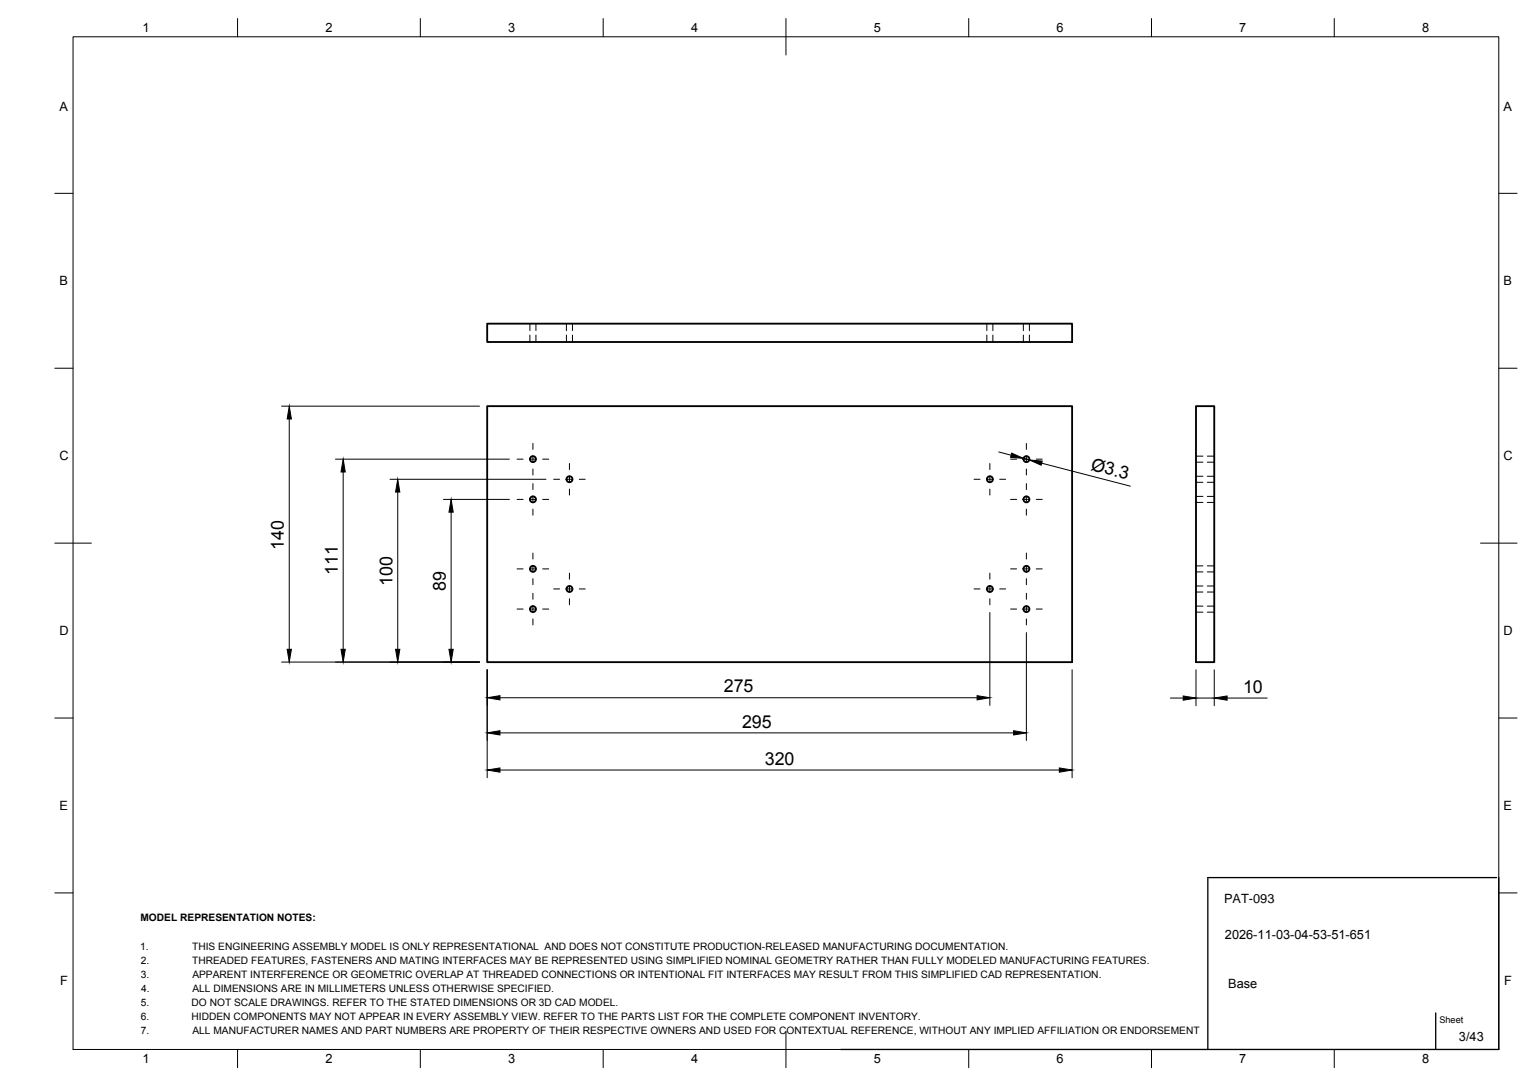
ISO-10303-21;
HEADER;
/* Generated by software containing ST-Developer
 * from STEP Tools, Inc. (www.steptools.com) 
 */

FILE_DESCRIPTION(
/* description */ ('Self-centering screw clamp'),
/* implementation_level */ '2;1');

FILE_NAME(
/* name */ 'Base.step',
/* time_stamp */ '2026-10-28T03:25:31-07:00',
/* author */ (''),
/* organization */ (''),
/* preprocessor_version */ 'ST-DEVELOPER v20.2',
/* originating_system */ 'Autodesk Translation Framework v15.17.0.0',
/* authorisation */ '');

FILE_SCHEMA (('AUTOMOTIVE_DESIGN { 1 0 10303 214 3 1 1 }'));
ENDSEC;

DATA;
#10=MECHANICAL_DESIGN_GEOMETRIC_PRESENTATION_REPRESENTATION('',(#624),#16799);
#542=SHAPE_REPRESENTATION_RELATIONSHIP('SRR','None',#17015,#583);
#583=ADVANCED_BREP_SHAPE_REPRESENTATION('',(#672),#16753);
#624=STYLED_ITEM('',(#17305),#672);
#672=MANIFOLD_SOLID_BREP('Body1',#9075);
#718=FACE_BOUND('',#1794,.T.);
#719=FACE_BOUND('',#1795,.T.);
#720=FACE_BOUND('',#1796,.T.);
#721=FACE_BOUND('',#1797,.T.);
#722=FACE_BOUND('',#1798,.T.);
#723=FACE_BOUND('',#1799,.T.);
#724=FACE_BOUND('',#1800,.T.);
#725=FACE_BOUND('',#1801,.T.);
#726=FACE_BOUND('',#1802,.T.);
#727=FACE_BOUND('',#1803,.T.);
#728=FACE_BOUND('',#1804,.T.);
#729=FACE_BOUND('',#1805,.T.);
#730=FACE_BOUND('',#1807,.T.);
#731=FACE_BOUND('',#1808,.T.);
#732=FACE_BOUND('',#1809,.T.);
#733=FACE_BOUND('',#1810,.T.);
#734=FACE_BOUND('',#1811,.T.);
#735=FACE_BOUND('',#1812,.T.);
#736=FACE_BOUND('',#1813,.T.);
#737=FACE_BOUND('',#1814,.T.);
#738=FACE_BOUND('',#1815,.T.);
#739=FACE_BOUND('',#1816,.T.);
#740=FACE_BOUND('',#1817,.T.);
#741=FACE_BOUND('',#1818,.T.);
#1014=PLANE('',#9616);
#1015=PLANE('',#9617);
#1016=PLANE('',#9618);
#1017=PLANE('',#9619);
#1018=PLANE('',#9620);
#1019=PLANE('',#9621);
#1273=FACE_OUTER_BOUND('',#1777,.T.);
#1274=FACE_OUTER_BOUND('',#1778,.T.);
#1275=FACE_OUTER_BOUND('',#1779,.T.);
#1276=FACE_OUTER_BOUND('',#1780,.T.);
#1277=FACE_OUTER_BOUND('',#1781,.T.);
#1278=FACE_OUTER_BOUND('',#1782,.T.);
#1279=FACE_OUTER_BOUND('',#1783,.T.);
#1280=FACE_OUTER_BOUND('',#1784,.T.);
#1281=FACE_OUTER_BOUND('',#1785,.T.);
#1282=FACE_OUTER_BOUND('',#1786,.T.);
#1283=FACE_OUTER_BOUND('',#1787,.T.);
#1284=FACE_OUTER_BOUND('',#1788,.T.);
#1285=FACE_OUTER_BOUND('',#1789,.T.);
#1286=FACE_OUTER_BOUND('',#1790,.T.);
#1287=FACE_OUTER_BOUND('',#1791,.T.);
#1288=FACE_OUTER_BOUND('',#1792,.T.);
#1289=FACE_OUTER_BOUND('',#1793,.T.);
#1290=FACE_OUTER_BOUND('',#1806,.T.);
#1777=EDGE_LOOP('',(#6103,#6104,#6105,#6106));
#1778=EDGE_LOOP('',(#6107,#6108,#6109,#6110));
#1779=EDGE_LOOP('',(#6111,#6112,#6113,#6114));
#1780=EDGE_LOOP('',(#6115,#6116,#6117,#6118));
#1781=EDGE_LOOP('',(#6119,#6120,#6121,#6122));
#1782=EDGE_LOOP('',(#6123,#6124,#6125,#6126));
#1783=EDGE_LOOP('',(#6127,#6128,#6129,#6130));
#1784=EDGE_LOOP('',(#6131,#6132,#6133,#6134));
#1785=EDGE_LOOP('',(#6135,#6136,#6137,#6138));
#1786=EDGE_LOOP('',(#6139,#6140,#6141,#6142));
#1787=EDGE_LOOP('',(#6143,#6144,#6145,#6146));
#1788=EDGE_LOOP('',(#6147,#6148,#6149,#6150));
#1789=EDGE_LOOP('',(#6151,#6152,#6153,#6154));
#1790=EDGE_LOOP('',(#6155,#6156,#6157,#6158));
#1791=EDGE_LOOP('',(#6159,#6160,#6161,#6162));
#1792=EDGE_LOOP('',(#6163,#6164,#6165,#6166));
#1793=EDGE_LOOP('',(#6167,#6168,#6169,#6170));
#1794=EDGE_LOOP('',(#6171));
#1795=EDGE_LOOP('',(#6172));
#1796=EDGE_LOOP('',(#6173));
#1797=EDGE_LOOP('',(#6174));
#1798=EDGE_LOOP('',(#6175));
#1799=EDGE_LOOP('',(#6176));
#1800=EDGE_LOOP('',(#6177));
#1801=EDGE_LOOP('',(#6178));
#1802=EDGE_LOOP('',(#6179));
#1803=EDGE_LOOP('',(#6180));
#1804=EDGE_LOOP('',(#6181));
#1805=EDGE_LOOP('',(#6182));
#1806=EDGE_LOOP('',(#6183,#6184,#6185,#6186));
#1807=EDGE_LOOP('',(#6187));
#1808=EDGE_LOOP('',(#6188));
#1809=EDGE_LOOP('',(#6189));
#1810=EDGE_LOOP('',(#6190));
#1811=EDGE_LOOP('',(#6191));
#1812=EDGE_LOOP('',(#6192));
#1813=EDGE_LOOP('',(#6193));
#1814=EDGE_LOOP('',(#6194));
#1815=EDGE_LOOP('',(#6195));
#1816=EDGE_LOOP('',(#6196));
#1817=EDGE_LOOP('',(#6197));
#1818=EDGE_LOOP('',(#6198));
#2577=LINE('',#13682,#3150);
#2578=LINE('',#13688,#3151);
#2579=LINE('',#13694,#3152);
#2580=LINE('',#13700,#3153);
#2581=LINE('',#13706,#3154);
#2582=LINE('',#13712,#3155);
#2583=LINE('',#13718,#3156);
#2584=LINE('',#13724,#3157);
#2585=LINE('',#13730,#3158);
#2586=LINE('',#13736,#3159);
#2587=LINE('',#13742,#3160);
#2588=LINE('',#13748,#3161);
#2589=LINE('',#13753,#3162);
#2590=LINE('',#13755,#3163);
#2591=LINE('',#13757,#3164);
#2592=LINE('',#13758,#3165);
#2593=LINE('',#13761,#3166);
#2594=LINE('',#13763,#3167);
#2595=LINE('',#13764,#3168);
#2596=LINE('',#13767,#3169);
#2597=LINE('',#13769,#3170);
#2598=LINE('',#13770,#3171);
#2599=LINE('',#13772,#3172);
#2600=LINE('',#13773,#3173);
#3150=VECTOR('',#10762,0.164999999999999);
#3151=VECTOR('',#10769,0.164999999999999);
#3152=VECTOR('',#10776,0.164999999999999);
#3153=VECTOR('',#10783,0.164999999999999);
#3154=VECTOR('',#10790,0.164999999999999);
#3155=VECTOR('',#10797,0.164999999999999);
#3156=VECTOR('',#10804,0.164999999999999);
#3157=VECTOR('',#10811,0.164999999999999);
#3158=VECTOR('',#10818,0.164999999999999);
#3159=VECTOR('',#10825,0.164999999999999);
#3160=VECTOR('',#10832,0.164999999999999);
#3161=VECTOR('',#10839,0.164999999999999);
#3162=VECTOR('',#10844,1.);
#3163=VECTOR('',#10845,1.);
#3164=VECTOR('',#10846,1.);
#3165=VECTOR('',#10847,1.);
#3166=VECTOR('',#10850,1.);
#3167=VECTOR('',#10851,1.);
#3168=VECTOR('',#10852,1.);
#3169=VECTOR('',#10855,1.);
#3170=VECTOR('',#10856,1.);
#3171=VECTOR('',#10857,1.);
#3172=VECTOR('',#10860,1.);
#3173=VECTOR('',#10861,1.);
#3723=CIRCLE('',#9581,0.164999999999999);
#3724=CIRCLE('',#9582,0.164999999999999);
#3725=CIRCLE('',#9584,0.164999999999999);
#3726=CIRCLE('',#9585,0.164999999999999);
#3727=CIRCLE('',#9587,0.164999999999999);
#3728=CIRCLE('',#9588,0.164999999999999);
#3729=CIRCLE('',#9590,0.164999999999999);
#3730=CIRCLE('',#9591,0.164999999999999);
#3731=CIRCLE('',#9593,0.164999999999999);
#3732=CIRCLE('',#9594,0.164999999999999);
#3733=CIRCLE('',#9596,0.164999999999999);
#3734=CIRCLE('',#9597,0.164999999999999);
#3735=CIRCLE('',#9599,0.164999999999999);
#3736=CIRCLE('',#9600,0.164999999999999);
#3737=CIRCLE('',#9602,0.164999999999999);
#3738=CIRCLE('',#9603,0.164999999999999);
#3739=CIRCLE('',#9605,0.164999999999999);
#3740=CIRCLE('',#9606,0.164999999999999);
#3741=CIRCLE('',#9608,0.164999999999999);
#3742=CIRCLE('',#9609,0.164999999999999);
#3743=CIRCLE('',#9611,0.164999999999999);
#3744=CIRCLE('',#9612,0.164999999999999);
#3745=CIRCLE('',#9614,0.164999999999999);
#3746=CIRCLE('',#9615,0.164999999999999);
#4233=VERTEX_POINT('',#13679);
#4234=VERTEX_POINT('',#13681);
#4235=VERTEX_POINT('',#13685);
#4236=VERTEX_POINT('',#13687);
#4237=VERTEX_POINT('',#13691);
#4238=VERTEX_POINT('',#13693);
#4239=VERTEX_POINT('',#13697);
#4240=VERTEX_POINT('',#13699);
#4241=VERTEX_POINT('',#13703);
#4242=VERTEX_POINT('',#13705);
#4243=VERTEX_POINT('',#13709);
#4244=VERTEX_POINT('',#13711);
#4245=VERTEX_POINT('',#13715);
#4246=VERTEX_POINT('',#13717);
#4247=VERTEX_POINT('',#13721);
#4248=VERTEX_POINT('',#13723);
#4249=VERTEX_POINT('',#13727);
#4250=VERTEX_POINT('',#13729);
#4251=VERTEX_POINT('',#13733);
#4252=VERTEX_POINT('',#13735);
#4253=VERTEX_POINT('',#13739);
#4254=VERTEX_POINT('',#13741);
#4255=VERTEX_POINT('',#13745);
#4256=VERTEX_POINT('',#13747);
#4257=VERTEX_POINT('',#13751);
#4258=VERTEX_POINT('',#13752);
#4259=VERTEX_POINT('',#13754);
#4260=VERTEX_POINT('',#13756);
#4261=VERTEX_POINT('',#13760);
#4262=VERTEX_POINT('',#13762);
#4263=VERTEX_POINT('',#13766);
#4264=VERTEX_POINT('',#13768);
#4976=EDGE_CURVE('',#4233,#4233,#3723,.T.);
#4977=EDGE_CURVE('',#4233,#4234,#2577,.T.);
#4978=EDGE_CURVE('',#4234,#4234,#3724,.T.);
#4979=EDGE_CURVE('',#4235,#4235,#3725,.T.);
#4980=EDGE_CURVE('',#4235,#4236,#2578,.T.);
#4981=EDGE_CURVE('',#4236,#4236,#3726,.T.);
#4982=EDGE_CURVE('',#4237,#4237,#3727,.T.);
#4983=EDGE_CURVE('',#4237,#4238,#2579,.T.);
#4984=EDGE_CURVE('',#4238,#4238,#3728,.T.);
#4985=EDGE_CURVE('',#4239,#4239,#3729,.T.);
#4986=EDGE_CURVE('',#4239,#4240,#2580,.T.);
#4987=EDGE_CURVE('',#4240,#4240,#3730,.T.);
#4988=EDGE_CURVE('',#4241,#4241,#3731,.T.);
#4989=EDGE_CURVE('',#4241,#4242,#2581,.T.);
#4990=EDGE_CURVE('',#4242,#4242,#3732,.T.);
#4991=EDGE_CURVE('',#4243,#4243,#3733,.T.);
#4992=EDGE_CURVE('',#4243,#4244,#2582,.T.);
#4993=EDGE_CURVE('',#4244,#4244,#3734,.T.);
#4994=EDGE_CURVE('',#4245,#4245,#3735,.T.);
#4995=EDGE_CURVE('',#4245,#4246,#2583,.T.);
#4996=EDGE_CURVE('',#4246,#4246,#3736,.T.);
#4997=EDGE_CURVE('',#4247,#4247,#3737,.T.);
#4998=EDGE_CURVE('',#4247,#4248,#2584,.T.);
#4999=EDGE_CURVE('',#4248,#4248,#3738,.T.);
#5000=EDGE_CURVE('',#4249,#4249,#3739,.T.);
#5001=EDGE_CURVE('',#4249,#4250,#2585,.T.);
#5002=EDGE_CURVE('',#4250,#4250,#3740,.T.);
#5003=EDGE_CURVE('',#4251,#4251,#3741,.T.);
#5004=EDGE_CURVE('',#4251,#4252,#2586,.T.);
#5005=EDGE_CURVE('',#4252,#4252,#3742,.T.);
#5006=EDGE_CURVE('',#4253,#4253,#3743,.T.);
#5007=EDGE_CURVE('',#4253,#4254,#2587,.T.);
#5008=EDGE_CURVE('',#4254,#4254,#3744,.T.);
#5009=EDGE_CURVE('',#4255,#4255,#3745,.T.);
#5010=EDGE_CURVE('',#4255,#4256,#2588,.T.);
#5011=EDGE_CURVE('',#4256,#4256,#3746,.T.);
#5012=EDGE_CURVE('',#4257,#4258,#2589,.T.);
#5013=EDGE_CURVE('',#4258,#4259,#2590,.T.);
#5014=EDGE_CURVE('',#4260,#4259,#2591,.T.);
#5015=EDGE_CURVE('',#4257,#4260,#2592,.T.);
#5016=EDGE_CURVE('',#4261,#4257,#2593,.T.);
#5017=EDGE_CURVE('',#4262,#4260,#2594,.T.);
#5018=EDGE_CURVE('',#4261,#4262,#2595,.T.);
#5019=EDGE_CURVE('',#4263,#4261,#2596,.T.);
#5020=EDGE_CURVE('',#4264,#4262,#2597,.T.);
#5021=EDGE_CURVE('',#4263,#4264,#2598,.T.);
#5022=EDGE_CURVE('',#4258,#4263,#2599,.T.);
#5023=EDGE_CURVE('',#4259,#4264,#2600,.T.);
#6103=ORIENTED_EDGE('',*,*,#4976,.F.);
#6104=ORIENTED_EDGE('',*,*,#4977,.T.);
#6105=ORIENTED_EDGE('',*,*,#4978,.F.);
#6106=ORIENTED_EDGE('',*,*,#4977,.F.);
#6107=ORIENTED_EDGE('',*,*,#4979,.F.);
#6108=ORIENTED_EDGE('',*,*,#4980,.T.);
#6109=ORIENTED_EDGE('',*,*,#4981,.F.);
#6110=ORIENTED_EDGE('',*,*,#4980,.F.);
#6111=ORIENTED_EDGE('',*,*,#4982,.F.);
#6112=ORIENTED_EDGE('',*,*,#4983,.T.);
#6113=ORIENTED_EDGE('',*,*,#4984,.F.);
#6114=ORIENTED_EDGE('',*,*,#4983,.F.);
#6115=ORIENTED_EDGE('',*,*,#4985,.F.);
#6116=ORIENTED_EDGE('',*,*,#4986,.T.);
#6117=ORIENTED_EDGE('',*,*,#4987,.F.);
#6118=ORIENTED_EDGE('',*,*,#4986,.F.);
#6119=ORIENTED_EDGE('',*,*,#4988,.F.);
#6120=ORIENTED_EDGE('',*,*,#4989,.T.);
#6121=ORIENTED_EDGE('',*,*,#4990,.F.);
#6122=ORIENTED_EDGE('',*,*,#4989,.F.);
#6123=ORIENTED_EDGE('',*,*,#4991,.F.);
#6124=ORIENTED_EDGE('',*,*,#4992,.T.);
#6125=ORIENTED_EDGE('',*,*,#4993,.F.);
#6126=ORIENTED_EDGE('',*,*,#4992,.F.);
#6127=ORIENTED_EDGE('',*,*,#4994,.F.);
#6128=ORIENTED_EDGE('',*,*,#4995,.T.);
#6129=ORIENTED_EDGE('',*,*,#4996,.F.);
#6130=ORIENTED_EDGE('',*,*,#4995,.F.);
#6131=ORIENTED_EDGE('',*,*,#4997,.F.);
#6132=ORIENTED_EDGE('',*,*,#4998,.T.);
#6133=ORIENTED_EDGE('',*,*,#4999,.F.);
#6134=ORIENTED_EDGE('',*,*,#4998,.F.);
#6135=ORIENTED_EDGE('',*,*,#5000,.F.);
#6136=ORIENTED_EDGE('',*,*,#5001,.T.);
#6137=ORIENTED_EDGE('',*,*,#5002,.F.);
#6138=ORIENTED_EDGE('',*,*,#5001,.F.);
#6139=ORIENTED_EDGE('',*,*,#5003,.F.);
#6140=ORIENTED_EDGE('',*,*,#5004,.T.);
#6141=ORIENTED_EDGE('',*,*,#5005,.F.);
#6142=ORIENTED_EDGE('',*,*,#5004,.F.);
#6143=ORIENTED_EDGE('',*,*,#5006,.F.);
#6144=ORIENTED_EDGE('',*,*,#5007,.T.);
#6145=ORIENTED_EDGE('',*,*,#5008,.F.);
#6146=ORIENTED_EDGE('',*,*,#5007,.F.);
#6147=ORIENTED_EDGE('',*,*,#5009,.F.);
#6148=ORIENTED_EDGE('',*,*,#5010,.T.);
#6149=ORIENTED_EDGE('',*,*,#5011,.F.);
#6150=ORIENTED_EDGE('',*,*,#5010,.F.);
#6151=ORIENTED_EDGE('',*,*,#5012,.T.);
#6152=ORIENTED_EDGE('',*,*,#5013,.T.);
#6153=ORIENTED_EDGE('',*,*,#5014,.F.);
#6154=ORIENTED_EDGE('',*,*,#5015,.F.);
#6155=ORIENTED_EDGE('',*,*,#5016,.T.);
#6156=ORIENTED_EDGE('',*,*,#5015,.T.);
#6157=ORIENTED_EDGE('',*,*,#5017,.F.);
#6158=ORIENTED_EDGE('',*,*,#5018,.F.);
#6159=ORIENTED_EDGE('',*,*,#5019,.T.);
#6160=ORIENTED_EDGE('',*,*,#5018,.T.);
#6161=ORIENTED_EDGE('',*,*,#5020,.F.);
#6162=ORIENTED_EDGE('',*,*,#5021,.F.);
#6163=ORIENTED_EDGE('',*,*,#5022,.T.);
#6164=ORIENTED_EDGE('',*,*,#5021,.T.);
#6165=ORIENTED_EDGE('',*,*,#5023,.F.);
#6166=ORIENTED_EDGE('',*,*,#5013,.F.);
#6167=ORIENTED_EDGE('',*,*,#5023,.T.);
#6168=ORIENTED_EDGE('',*,*,#5020,.T.);
#6169=ORIENTED_EDGE('',*,*,#5017,.T.);
#6170=ORIENTED_EDGE('',*,*,#5014,.T.);
#6171=ORIENTED_EDGE('',*,*,#4984,.T.);
#6172=ORIENTED_EDGE('',*,*,#4987,.T.);
#6173=ORIENTED_EDGE('',*,*,#5011,.T.);
#6174=ORIENTED_EDGE('',*,*,#5008,.T.);
#6175=ORIENTED_EDGE('',*,*,#5005,.T.);
#6176=ORIENTED_EDGE('',*,*,#5002,.T.);
#6177=ORIENTED_EDGE('',*,*,#4999,.T.);
#6178=ORIENTED_EDGE('',*,*,#4996,.T.);
#6179=ORIENTED_EDGE('',*,*,#4993,.T.);
#6180=ORIENTED_EDGE('',*,*,#4990,.T.);
#6181=ORIENTED_EDGE('',*,*,#4981,.T.);
#6182=ORIENTED_EDGE('',*,*,#4978,.T.);
#6183=ORIENTED_EDGE('',*,*,#5022,.F.);
#6184=ORIENTED_EDGE('',*,*,#5012,.F.);
#6185=ORIENTED_EDGE('',*,*,#5016,.F.);
#6186=ORIENTED_EDGE('',*,*,#5019,.F.);
#6187=ORIENTED_EDGE('',*,*,#4982,.T.);
#6188=ORIENTED_EDGE('',*,*,#4985,.T.);
#6189=ORIENTED_EDGE('',*,*,#5009,.T.);
#6190=ORIENTED_EDGE('',*,*,#5006,.T.);
#6191=ORIENTED_EDGE('',*,*,#5003,.T.);
#6192=ORIENTED_EDGE('',*,*,#5000,.T.);
#6193=ORIENTED_EDGE('',*,*,#4997,.T.);
#6194=ORIENTED_EDGE('',*,*,#4994,.T.);
#6195=ORIENTED_EDGE('',*,*,#4991,.T.);
#6196=ORIENTED_EDGE('',*,*,#4988,.T.);
#6197=ORIENTED_EDGE('',*,*,#4979,.T.);
#6198=ORIENTED_EDGE('',*,*,#4976,.T.);
#8357=CYLINDRICAL_SURFACE('',#9580,0.164999999999999);
#8358=CYLINDRICAL_SURFACE('',#9583,0.164999999999999);
#8359=CYLINDRICAL_SURFACE('',#9586,0.164999999999999);
#8360=CYLINDRICAL_SURFACE('',#9589,0.164999999999999);
#8361=CYLINDRICAL_SURFACE('',#9592,0.164999999999999);
#8362=CYLINDRICAL_SURFACE('',#9595,0.164999999999999);
#8363=CYLINDRICAL_SURFACE('',#9598,0.164999999999999);
#8364=CYLINDRICAL_SURFACE('',#9601,0.164999999999999);
#8365=CYLINDRICAL_SURFACE('',#9604,0.164999999999999);
#8366=CYLINDRICAL_SURFACE('',#9607,0.164999999999999);
#8367=CYLINDRICAL_SURFACE('',#9610,0.164999999999999);
#8368=CYLINDRICAL_SURFACE('',#9613,0.164999999999999);
#8571=ADVANCED_FACE('',(#1273),#8357,.F.);
#8572=ADVANCED_FACE('',(#1274),#8358,.F.);
#8573=ADVANCED_FACE('',(#1275),#8359,.F.);
#8574=ADVANCED_FACE('',(#1276),#8360,.F.);
#8575=ADVANCED_FACE('',(#1277),#8361,.F.);
#8576=ADVANCED_FACE('',(#1278),#8362,.F.);
#8577=ADVANCED_FACE('',(#1279),#8363,.F.);
#8578=ADVANCED_FACE('',(#1280),#8364,.F.);
#8579=ADVANCED_FACE('',(#1281),#8365,.F.);
#8580=ADVANCED_FACE('',(#1282),#8366,.F.);
#8581=ADVANCED_FACE('',(#1283),#8367,.F.);
#8582=ADVANCED_FACE('',(#1284),#8368,.F.);
#8583=ADVANCED_FACE('',(#1285),#1014,.T.);
#8584=ADVANCED_FACE('',(#1286),#1015,.T.);
#8585=ADVANCED_FACE('',(#1287),#1016,.T.);
#8586=ADVANCED_FACE('',(#1288),#1017,.T.);
#8587=ADVANCED_FACE('',(#1289,#718,#719,#720,#721,#722,#723,#724,#725,#726,
#727,#728,#729),#1018,.T.);
#8588=ADVANCED_FACE('',(#1290,#730,#731,#732,#733,#734,#735,#736,#737,#738,
#739,#740,#741),#1019,.F.);
#9075=CLOSED_SHELL('',(#8571,#8572,#8573,#8574,#8575,#8576,#8577,#8578,
#8579,#8580,#8581,#8582,#8583,#8584,#8585,#8586,#8587,#8588));
#9579=AXIS2_PLACEMENT_3D('',#13677,#10756,#10757);
#9580=AXIS2_PLACEMENT_3D('',#13678,#10758,#10759);
#9581=AXIS2_PLACEMENT_3D('',#13680,#10760,#10761);
#9582=AXIS2_PLACEMENT_3D('',#13683,#10763,#10764);
#9583=AXIS2_PLACEMENT_3D('',#13684,#10765,#10766);
#9584=AXIS2_PLACEMENT_3D('',#13686,#10767,#10768);
#9585=AXIS2_PLACEMENT_3D('',#13689,#10770,#10771);
#9586=AXIS2_PLACEMENT_3D('',#13690,#10772,#10773);
#9587=AXIS2_PLACEMENT_3D('',#13692,#10774,#10775);
#9588=AXIS2_PLACEMENT_3D('',#13695,#10777,#10778);
#9589=AXIS2_PLACEMENT_3D('',#13696,#10779,#10780);
#9590=AXIS2_PLACEMENT_3D('',#13698,#10781,#10782);
#9591=AXIS2_PLACEMENT_3D('',#13701,#10784,#10785);
#9592=AXIS2_PLACEMENT_3D('',#13702,#10786,#10787);
#9593=AXIS2_PLACEMENT_3D('',#13704,#10788,#10789);
#9594=AXIS2_PLACEMENT_3D('',#13707,#10791,#10792);
#9595=AXIS2_PLACEMENT_3D('',#13708,#10793,#10794);
#9596=AXIS2_PLACEMENT_3D('',#13710,#10795,#10796);
#9597=AXIS2_PLACEMENT_3D('',#13713,#10798,#10799);
#9598=AXIS2_PLACEMENT_3D('',#13714,#10800,#10801);
#9599=AXIS2_PLACEMENT_3D('',#13716,#10802,#10803);
#9600=AXIS2_PLACEMENT_3D('',#13719,#10805,#10806);
#9601=AXIS2_PLACEMENT_3D('',#13720,#10807,#10808);
#9602=AXIS2_PLACEMENT_3D('',#13722,#10809,#10810);
#9603=AXIS2_PLACEMENT_3D('',#13725,#10812,#10813);
#9604=AXIS2_PLACEMENT_3D('',#13726,#10814,#10815);
#9605=AXIS2_PLACEMENT_3D('',#13728,#10816,#10817);
#9606=AXIS2_PLACEMENT_3D('',#13731,#10819,#10820);
#9607=AXIS2_PLACEMENT_3D('',#13732,#10821,#10822);
#9608=AXIS2_PLACEMENT_3D('',#13734,#10823,#10824);
#9609=AXIS2_PLACEMENT_3D('',#13737,#10826,#10827);
#9610=AXIS2_PLACEMENT_3D('',#13738,#10828,#10829);
#9611=AXIS2_PLACEMENT_3D('',#13740,#10830,#10831);
#9612=AXIS2_PLACEMENT_3D('',#13743,#10833,#10834);
#9613=AXIS2_PLACEMENT_3D('',#13744,#10835,#10836);
#9614=AXIS2_PLACEMENT_3D('',#13746,#10837,#10838);
#9615=AXIS2_PLACEMENT_3D('',#13749,#10840,#10841);
#9616=AXIS2_PLACEMENT_3D('',#13750,#10842,#10843);
#9617=AXIS2_PLACEMENT_3D('',#13759,#10848,#10849);
#9618=AXIS2_PLACEMENT_3D('',#13765,#10853,#10854);
#9619=AXIS2_PLACEMENT_3D('',#13771,#10858,#10859);
#9620=AXIS2_PLACEMENT_3D('',#13774,#10862,#10863);
#9621=AXIS2_PLACEMENT_3D('',#13775,#10864,#10865);
#10756=DIRECTION('axis',(0.,0.,1.));
#10757=DIRECTION('refdir',(1.,0.,0.));
#10758=DIRECTION('center_axis',(0.,0.,1.));
#10759=DIRECTION('ref_axis',(1.,0.,0.));
#10760=DIRECTION('center_axis',(0.,0.,1.));
#10761=DIRECTION('ref_axis',(1.,0.,0.));
#10762=DIRECTION('',(0.,0.,1.));
#10763=DIRECTION('center_axis',(0.,0.,-1.));
#10764=DIRECTION('ref_axis',(1.,0.,0.));
#10765=DIRECTION('center_axis',(0.,0.,1.));
#10766=DIRECTION('ref_axis',(1.,0.,0.));
#10767=DIRECTION('center_axis',(0.,0.,1.));
#10768=DIRECTION('ref_axis',(1.,0.,0.));
#10769=DIRECTION('',(0.,0.,1.));
#10770=DIRECTION('center_axis',(0.,0.,-1.));
#10771=DIRECTION('ref_axis',(1.,0.,0.));
#10772=DIRECTION('center_axis',(0.,0.,1.));
#10773=DIRECTION('ref_axis',(1.,0.,0.));
#10774=DIRECTION('center_axis',(0.,0.,1.));
#10775=DIRECTION('ref_axis',(1.,0.,0.));
#10776=DIRECTION('',(0.,0.,1.));
#10777=DIRECTION('center_axis',(0.,0.,-1.));
#10778=DIRECTION('ref_axis',(1.,0.,0.));
#10779=DIRECTION('center_axis',(0.,0.,1.));
#10780=DIRECTION('ref_axis',(1.,0.,0.));
#10781=DIRECTION('center_axis',(0.,0.,1.));
#10782=DIRECTION('ref_axis',(1.,0.,0.));
#10783=DIRECTION('',(0.,0.,1.));
#10784=DIRECTION('center_axis',(0.,0.,-1.));
#10785=DIRECTION('ref_axis',(1.,0.,0.));
#10786=DIRECTION('center_axis',(0.,0.,1.));
#10787=DIRECTION('ref_axis',(1.,0.,0.));
#10788=DIRECTION('center_axis',(0.,0.,1.));
#10789=DIRECTION('ref_axis',(1.,0.,0.));
#10790=DIRECTION('',(0.,0.,1.));
#10791=DIRECTION('center_axis',(0.,0.,-1.));
#10792=DIRECTION('ref_axis',(1.,0.,0.));
#10793=DIRECTION('center_axis',(0.,0.,1.));
#10794=DIRECTION('ref_axis',(1.,0.,0.));
#10795=DIRECTION('center_axis',(0.,0.,1.));
#10796=DIRECTION('ref_axis',(1.,0.,0.));
#10797=DIRECTION('',(0.,0.,1.));
#10798=DIRECTION('center_axis',(0.,0.,-1.));
#10799=DIRECTION('ref_axis',(1.,0.,0.));
#10800=DIRECTION('center_axis',(0.,0.,1.));
#10801=DIRECTION('ref_axis',(1.,0.,0.));
#10802=DIRECTION('center_axis',(0.,0.,1.));
#10803=DIRECTION('ref_axis',(1.,0.,0.));
#10804=DIRECTION('',(0.,0.,1.));
#10805=DIRECTION('center_axis',(0.,0.,-1.));
#10806=DIRECTION('ref_axis',(1.,0.,0.));
#10807=DIRECTION('center_axis',(0.,0.,1.));
#10808=DIRECTION('ref_axis',(1.,0.,0.));
#10809=DIRECTION('center_axis',(0.,0.,1.));
#10810=DIRECTION('ref_axis',(1.,0.,0.));
#10811=DIRECTION('',(0.,0.,1.));
#10812=DIRECTION('center_axis',(0.,0.,-1.));
#10813=DIRECTION('ref_axis',(1.,0.,0.));
#10814=DIRECTION('center_axis',(0.,0.,1.));
#10815=DIRECTION('ref_axis',(1.,0.,0.));
#10816=DIRECTION('center_axis',(0.,0.,1.));
#10817=DIRECTION('ref_axis',(1.,0.,0.));
#10818=DIRECTION('',(0.,0.,1.));
#10819=DIRECTION('center_axis',(0.,0.,-1.));
#10820=DIRECTION('ref_axis',(1.,0.,0.));
#10821=DIRECTION('center_axis',(0.,0.,1.));
#10822=DIRECTION('ref_axis',(1.,0.,0.));
#10823=DIRECTION('center_axis',(0.,0.,1.));
#10824=DIRECTION('ref_axis',(1.,0.,0.));
#10825=DIRECTION('',(0.,0.,1.));
#10826=DIRECTION('center_axis',(0.,0.,-1.));
#10827=DIRECTION('ref_axis',(1.,0.,0.));
#10828=DIRECTION('center_axis',(0.,0.,1.));
#10829=DIRECTION('ref_axis',(1.,0.,0.));
#10830=DIRECTION('center_axis',(0.,0.,1.));
#10831=DIRECTION('ref_axis',(1.,0.,0.));
#10832=DIRECTION('',(0.,0.,1.));
#10833=DIRECTION('center_axis',(0.,0.,-1.));
#10834=DIRECTION('ref_axis',(1.,0.,0.));
#10835=DIRECTION('center_axis',(0.,0.,1.));
#10836=DIRECTION('ref_axis',(1.,0.,0.));
#10837=DIRECTION('center_axis',(0.,0.,1.));
#10838=DIRECTION('ref_axis',(1.,0.,0.));
#10839=DIRECTION('',(0.,0.,1.));
#10840=DIRECTION('center_axis',(0.,0.,-1.));
#10841=DIRECTION('ref_axis',(1.,0.,0.));
#10842=DIRECTION('center_axis',(0.,1.,0.));
#10843=DIRECTION('ref_axis',(-1.,0.,0.));
#10844=DIRECTION('',(-1.,0.,0.));
#10845=DIRECTION('',(0.,0.,1.));
#10846=DIRECTION('',(-1.,0.,0.));
#10847=DIRECTION('',(0.,0.,1.));
#10848=DIRECTION('center_axis',(1.,0.,0.));
#10849=DIRECTION('ref_axis',(0.,1.,0.));
#10850=DIRECTION('',(0.,1.,0.));
#10851=DIRECTION('',(0.,1.,0.));
#10852=DIRECTION('',(0.,0.,1.));
#10853=DIRECTION('center_axis',(0.,-1.,0.));
#10854=DIRECTION('ref_axis',(1.,0.,0.));
#10855=DIRECTION('',(1.,0.,0.));
#10856=DIRECTION('',(1.,0.,0.));
#10857=DIRECTION('',(0.,0.,1.));
#10858=DIRECTION('center_axis',(-1.,0.,0.));
#10859=DIRECTION('ref_axis',(0.,-1.,0.));
#10860=DIRECTION('',(0.,-1.,0.));
#10861=DIRECTION('',(0.,-1.,0.));
#10862=DIRECTION('center_axis',(0.,0.,1.));
#10863=DIRECTION('ref_axis',(1.,0.,0.));
#10864=DIRECTION('center_axis',(0.,0.,1.));
#10865=DIRECTION('ref_axis',(1.,0.,0.));
#13677=CARTESIAN_POINT('',(0.,0.,0.));
#13678=CARTESIAN_POINT('Origin',(11.5,-3.,-0.1));
#13679=CARTESIAN_POINT('',(11.335,-3.,0.));
#13680=CARTESIAN_POINT('Origin',(11.5,-3.,0.));
#13681=CARTESIAN_POINT('',(11.335,-3.,1.));
#13682=CARTESIAN_POINT('',(11.335,-3.,-0.1));
#13683=CARTESIAN_POINT('Origin',(11.5,-3.,1.));
#13684=CARTESIAN_POINT('Origin',(11.5,3.,-0.1));
#13685=CARTESIAN_POINT('',(11.335,3.,0.));
#13686=CARTESIAN_POINT('Origin',(11.5,3.,0.));
#13687=CARTESIAN_POINT('',(11.335,3.,1.));
#13688=CARTESIAN_POINT('',(11.335,3.,-0.1));
#13689=CARTESIAN_POINT('Origin',(11.5,3.,1.));
#13690=CARTESIAN_POINT('Origin',(-11.5,-3.,-0.1));
#13691=CARTESIAN_POINT('',(-11.665,-3.,0.));
#13692=CARTESIAN_POINT('Origin',(-11.5,-3.,0.));
#13693=CARTESIAN_POINT('',(-11.665,-3.,1.));
#13694=CARTESIAN_POINT('',(-11.665,-3.,-0.1));
#13695=CARTESIAN_POINT('Origin',(-11.5,-3.,1.));
#13696=CARTESIAN_POINT('Origin',(-11.5,3.,-0.1));
#13697=CARTESIAN_POINT('',(-11.665,3.,0.));
#13698=CARTESIAN_POINT('Origin',(-11.5,3.,0.));
#13699=CARTESIAN_POINT('',(-11.665,3.,1.));
#13700=CARTESIAN_POINT('',(-11.665,3.,-0.1));
#13701=CARTESIAN_POINT('Origin',(-11.5,3.,1.));
#13702=CARTESIAN_POINT('Origin',(13.5,1.9,-0.1));
#13703=CARTESIAN_POINT('',(13.335,1.9,0.));
#13704=CARTESIAN_POINT('Origin',(13.5,1.9,0.));
#13705=CARTESIAN_POINT('',(13.335,1.9,1.));
#13706=CARTESIAN_POINT('',(13.335,1.9,-0.1));
#13707=CARTESIAN_POINT('Origin',(13.5,1.9,1.));
#13708=CARTESIAN_POINT('Origin',(13.5,4.1,-0.1));
#13709=CARTESIAN_POINT('',(13.335,4.1,0.));
#13710=CARTESIAN_POINT('Origin',(13.5,4.1,0.));
#13711=CARTESIAN_POINT('',(13.335,4.1,1.));
#13712=CARTESIAN_POINT('',(13.335,4.1,-0.1));
#13713=CARTESIAN_POINT('Origin',(13.5,4.1,1.));
#13714=CARTESIAN_POINT('Origin',(-13.5,1.9,-0.1));
#13715=CARTESIAN_POINT('',(-13.665,1.9,0.));
#13716=CARTESIAN_POINT('Origin',(-13.5,1.9,0.));
#13717=CARTESIAN_POINT('',(-13.665,1.9,1.));
#13718=CARTESIAN_POINT('',(-13.665,1.9,-0.1));
#13719=CARTESIAN_POINT('Origin',(-13.5,1.9,1.));
#13720=CARTESIAN_POINT('Origin',(-13.5,4.1,-0.1));
#13721=CARTESIAN_POINT('',(-13.665,4.1,0.));
#13722=CARTESIAN_POINT('Origin',(-13.5,4.1,0.));
#13723=CARTESIAN_POINT('',(-13.665,4.1,1.));
#13724=CARTESIAN_POINT('',(-13.665,4.1,-0.1));
#13725=CARTESIAN_POINT('Origin',(-13.5,4.1,1.));
#13726=CARTESIAN_POINT('Origin',(13.5,-4.1,-0.1));
#13727=CARTESIAN_POINT('',(13.335,-4.1,0.));
#13728=CARTESIAN_POINT('Origin',(13.5,-4.1,0.));
#13729=CARTESIAN_POINT('',(13.335,-4.1,1.));
#13730=CARTESIAN_POINT('',(13.335,-4.1,-0.1));
#13731=CARTESIAN_POINT('Origin',(13.5,-4.1,1.));
#13732=CARTESIAN_POINT('Origin',(13.5,-1.9,-0.1));
#13733=CARTESIAN_POINT('',(13.335,-1.9,0.));
#13734=CARTESIAN_POINT('Origin',(13.5,-1.9,0.));
#13735=CARTESIAN_POINT('',(13.335,-1.9,1.));
#13736=CARTESIAN_POINT('',(13.335,-1.9,-0.1));
#13737=CARTESIAN_POINT('Origin',(13.5,-1.9,1.));
#13738=CARTESIAN_POINT('Origin',(-13.5,-4.1,-0.1));
#13739=CARTESIAN_POINT('',(-13.665,-4.1,0.));
#13740=CARTESIAN_POINT('Origin',(-13.5,-4.1,0.));
#13741=CARTESIAN_POINT('',(-13.665,-4.1,1.));
#13742=CARTESIAN_POINT('',(-13.665,-4.1,-0.1));
#13743=CARTESIAN_POINT('Origin',(-13.5,-4.1,1.));
#13744=CARTESIAN_POINT('Origin',(-13.5,-1.9,-0.1));
#13745=CARTESIAN_POINT('',(-13.665,-1.9,0.));
#13746=CARTESIAN_POINT('Origin',(-13.5,-1.9,0.));
#13747=CARTESIAN_POINT('',(-13.665,-1.9,1.));
#13748=CARTESIAN_POINT('',(-13.665,-1.9,-0.1));
#13749=CARTESIAN_POINT('Origin',(-13.5,-1.9,1.));
#13750=CARTESIAN_POINT('Origin',(16.,7.,0.));
#13751=CARTESIAN_POINT('',(16.,7.,0.));
#13752=CARTESIAN_POINT('',(-16.,7.,0.));
#13753=CARTESIAN_POINT('',(16.,7.,0.));
#13754=CARTESIAN_POINT('',(-16.,7.,1.));
#13755=CARTESIAN_POINT('',(-16.,7.,0.));
#13756=CARTESIAN_POINT('',(16.,7.,1.));
#13757=CARTESIAN_POINT('',(16.,7.,1.));
#13758=CARTESIAN_POINT('',(16.,7.,0.));
#13759=CARTESIAN_POINT('Origin',(16.,-7.,0.));
#13760=CARTESIAN_POINT('',(16.,-7.,0.));
#13761=CARTESIAN_POINT('',(16.,-7.,0.));
#13762=CARTESIAN_POINT('',(16.,-7.,1.));
#13763=CARTESIAN_POINT('',(16.,-7.,1.));
#13764=CARTESIAN_POINT('',(16.,-7.,0.));
#13765=CARTESIAN_POINT('Origin',(-16.,-7.,0.));
#13766=CARTESIAN_POINT('',(-16.,-7.,0.));
#13767=CARTESIAN_POINT('',(-16.,-7.,0.));
#13768=CARTESIAN_POINT('',(-16.,-7.,1.));
#13769=CARTESIAN_POINT('',(-16.,-7.,1.));
#13770=CARTESIAN_POINT('',(-16.,-7.,0.));
#13771=CARTESIAN_POINT('Origin',(-16.,7.,0.));
#13772=CARTESIAN_POINT('',(-16.,7.,0.));
#13773=CARTESIAN_POINT('',(-16.,7.,1.));
#13774=CARTESIAN_POINT('Origin',(0.,0.,1.));
#13775=CARTESIAN_POINT('Origin',(0.,0.,0.));
#16704=UNCERTAINTY_MEASURE_WITH_UNIT(LENGTH_MEASURE(0.001),#16800,
'DISTANCE_ACCURACY_VALUE',
'Maximum model space distance between geometric entities at asserted c
onnectivities');
#16750=UNCERTAINTY_MEASURE_WITH_UNIT(LENGTH_MEASURE(0.001),#16800,
'DISTANCE_ACCURACY_VALUE',
'Maximum model space distance between geometric entities at asserted c
onnectivities');
#16753=(
GEOMETRIC_REPRESENTATION_CONTEXT(3)
GLOBAL_UNCERTAINTY_ASSIGNED_CONTEXT((#16704))
GLOBAL_UNIT_ASSIGNED_CONTEXT((#16800,#16802,#16803))
REPRESENTATION_CONTEXT('','3D')
);
#16799=(
GEOMETRIC_REPRESENTATION_CONTEXT(3)
GLOBAL_UNCERTAINTY_ASSIGNED_CONTEXT((#16750))
GLOBAL_UNIT_ASSIGNED_CONTEXT((#16800,#16802,#16803))
REPRESENTATION_CONTEXT('','3D')
);
#16800=(
LENGTH_UNIT()
NAMED_UNIT(*)
SI_UNIT(.CENTI.,.METRE.)
);
#16802=(
NAMED_UNIT(*)
PLANE_ANGLE_UNIT()
SI_UNIT($,.RADIAN.)
);
#16803=(
NAMED_UNIT(*)
SI_UNIT($,.STERADIAN.)
SOLID_ANGLE_UNIT()
);
#16806=SHAPE_DEFINITION_REPRESENTATION(#16854,#17015);
#16854=PRODUCT_DEFINITION_SHAPE('',$,#17064);
#17015=SHAPE_REPRESENTATION('',(#9579),#16753);
#17061=PRODUCT_DEFINITION_CONTEXT('part definition',#17207,'design');
#17064=PRODUCT_DEFINITION('Base','Base',#17112,#17061);
#17112=PRODUCT_DEFINITION_FORMATION('',$,#17211);
#17207=APPLICATION_CONTEXT(
'Core Data for Automotive Mechanical Design Process');
#17208=PRODUCT_CONTEXT('part definition',#17207,'mechanical');
#17211=PRODUCT('Base','Base','Base',(#17208));
#17299=COLOUR_RGB('Dark Blue',0.08,0.2,0.34);
#17300=FILL_AREA_STYLE_COLOUR('',#17299);
#17301=FILL_AREA_STYLE('',(#17300));
#17302=SURFACE_STYLE_FILL_AREA(#17301);
#17303=SURFACE_SIDE_STYLE('',(#17302));
#17304=SURFACE_STYLE_USAGE(.BOTH.,#17303);
#17305=PRESENTATION_STYLE_ASSIGNMENT((#17304));
ENDSEC;
END-ISO-10303-21;
